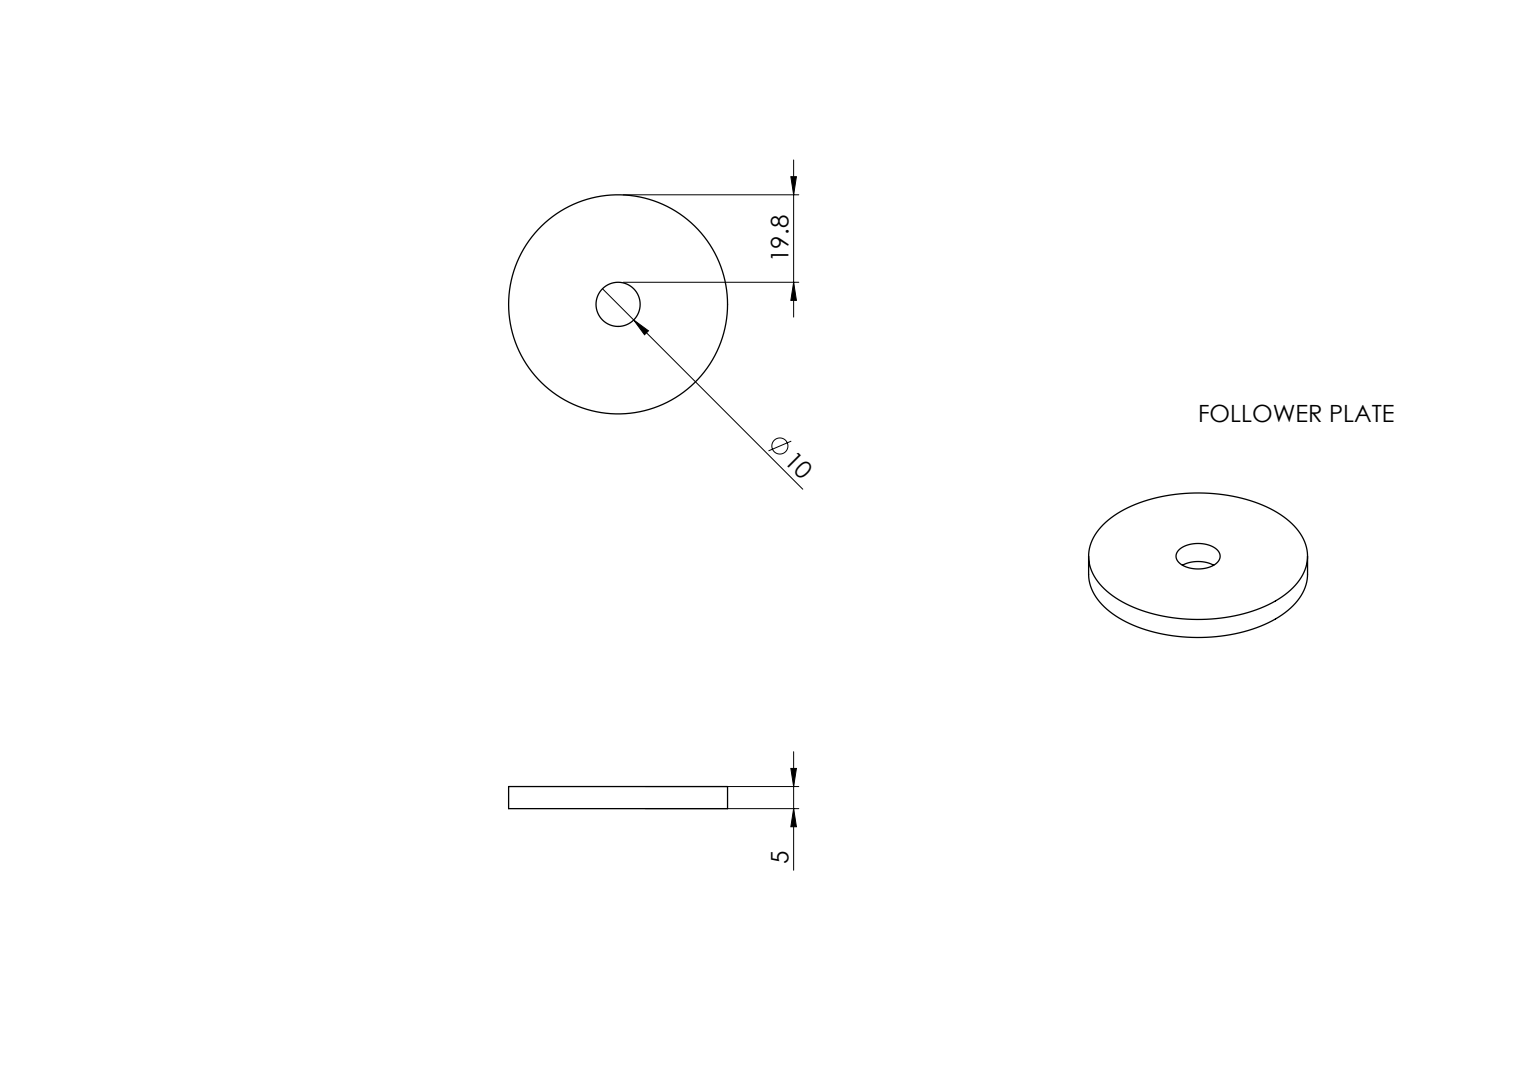
ISO-10303-21;
HEADER;
FILE_DESCRIPTION (('STEP AP214'),
    '1' );
FILE_NAME ('follower plate.step',
    '2026-10-31T03:36:27',
    ( '' ),
    ( '' ),
    'SwSTEP 2.0',
    'SolidWorks 2026',
    '' );
FILE_SCHEMA (( 'AUTOMOTIVE_DESIGN' ));
ENDSEC;

DATA;
#186=CARTESIAN_POINT ( 'NONE',  ( 0.000000000000000000, 148.0000000000000000, 0.000000000000000000 ) ) ;
#892=DIRECTION ( 'NONE',  ( 1.000000000000000000, 0.000000000000000000, 0.000000000000000000 ) ) ;
#1332=VECTOR ( 'NONE', #31249, 1000.000000000000000 ) ;
#1567=APPLICATION_CONTEXT ( 'automotive_design' ) ;
#1999=CLOSED_SHELL ( 'NONE', ( #16368, #12231, #10763, #12020, #10658, #28577 ) ) ;
#2419=AXIS2_PLACEMENT_3D ( 'NONE', #186, #17642, #35053 ) ;
#2606=ORIENTED_EDGE ( 'NONE', *, *, #4345, .F. ) ;
#2751=DIRECTION ( 'NONE',  ( 0.000000000000000000, 0.000000000000000000, -1.000000000000000000 ) ) ;
#3108=PRESENTATION_STYLE_ASSIGNMENT (( #5764 ) ) ;
#3154=CARTESIAN_POINT ( 'NONE',  ( 0.000000000000000000, 148.0000000000000000, -5.000000000000000888 ) ) ;
#3391=EDGE_CURVE ( 'NONE', #15520, #17083, #7946, .T. ) ;
#3436=AXIS2_PLACEMENT_3D ( 'NONE', #21969, #13622, #10578 ) ;
#3512=PRODUCT ( 'follower plate', 'follower plate', '', ( #4473 ) ) ;
#3678=EDGE_CURVE ( 'NONE', #35499, #36556, #26294, .T. ) ;
#3830=( GEOMETRIC_REPRESENTATION_CONTEXT ( 3 ) GLOBAL_UNCERTAINTY_ASSIGNED_CONTEXT ( ( #10847 ) ) GLOBAL_UNIT_ASSIGNED_CONTEXT ( ( #27171, #6708, #30204 ) ) REPRESENTATION_CONTEXT ( 'NONE', 'WORKASPACE' ) );
#4005=EDGE_CURVE ( 'NONE', #19287, #15548, #15251, .T. ) ;
#4007=ORIENTED_EDGE ( 'NONE', *, *, #23768, .F. ) ;
#4149=CIRCLE ( 'NONE', #8989, 5.000000000000000888 ) ;
#4345=EDGE_CURVE ( 'NONE', #35499, #15520, #10408, .T. ) ;
#4473=PRODUCT_CONTEXT ( 'NONE', #1567, 'mechanical' ) ;
#4527=SHAPE_REPRESENTATION ( 'follower plate', ( #17215 ), #16540 ) ;
#4651=DIRECTION ( 'NONE',  ( 0.000000000000000000, 0.000000000000000000, 1.000000000000000000 ) ) ;
#5261=CYLINDRICAL_SURFACE ( 'NONE', #3436, 5.000000000000000888 ) ;
#5315=LINE ( 'NONE', #16892, #20213 ) ;
#5752=ORIENTED_EDGE ( 'NONE', *, *, #7976, .F. ) ;
#5764=SURFACE_STYLE_USAGE ( .BOTH. , #34577 ) ;
#5780=CYLINDRICAL_SURFACE ( 'NONE', #25925, 24.80000000000000426 ) ;
#5837=CARTESIAN_POINT ( 'NONE',  ( 0.000000000000000000, 143.0000000000000000, 0.000000000000000000 ) ) ;
#5951=SURFACE_STYLE_FILL_AREA ( #23029 ) ;
#6046=CARTESIAN_POINT ( 'NONE',  ( 0.000000000000000000, 143.0000000000000000, -5.000000000000000888 ) ) ;
#6236=PRODUCT_DEFINITION_SHAPE ( 'NONE', 'NONE',  #37054 ) ;
#6285=DIRECTION ( 'NONE',  ( 0.000000000000000000, 0.000000000000000000, -1.000000000000000000 ) ) ;
#6655=ORIENTED_EDGE ( 'NONE', *, *, #4345, .T. ) ;
#6708=( NAMED_UNIT ( * ) PLANE_ANGLE_UNIT ( ) SI_UNIT ( $, .RADIAN. ) );
#6775=DIRECTION ( 'NONE',  ( 0.000000000000000000, 1.000000000000000000, 0.000000000000000000 ) ) ;
#7289=ORIENTED_EDGE ( 'NONE', *, *, #4005, .F. ) ;
#7513=MANIFOLD_SOLID_BREP ( 'Extrude-Thin1', #1999 ) ;
#7946=LINE ( 'NONE', #33719, #1332 ) ;
#7976=EDGE_CURVE ( 'NONE', #36216, #15548, #5315, .T. ) ;
#8069=COLOUR_RGB ( '',0.8941176470588234615, 0.8941176470588234615, 0.8941176470588234615 ) ;
#8268=FACE_OUTER_BOUND ( 'NONE', #23646, .T. ) ;
#8795=ORIENTED_EDGE ( 'NONE', *, *, #32424, .F. ) ;
#8806=( LENGTH_UNIT ( ) NAMED_UNIT ( * ) SI_UNIT ( .MILLI., .METRE. ) );
#8989=AXIS2_PLACEMENT_3D ( 'NONE', #29950, #18597, #33170 ) ;
#8991=( NAMED_UNIT ( * ) PLANE_ANGLE_UNIT ( ) SI_UNIT ( $, .RADIAN. ) );
#9205=EDGE_LOOP ( 'NONE', ( #23577, #31014, #20897, #8795 ) ) ;
#9458=CIRCLE ( 'NONE', #29444, 5.000000000000000888 ) ;
#9808=DIRECTION ( 'NONE',  ( -0.000000000000000000, -1.000000000000000000, -0.000000000000000000 ) ) ;
#9992=CARTESIAN_POINT ( 'NONE',  ( 0.000000000000000000, 148.0000000000000000, 0.000000000000000000 ) ) ;
#10237=ORIENTED_EDGE ( 'NONE', *, *, #3391, .T. ) ;
#10268=ORIENTED_EDGE ( 'NONE', *, *, #32424, .T. ) ;
#10369=CARTESIAN_POINT ( 'NONE',  ( 0.000000000000000000, 148.0000000000000000, 0.000000000000000000 ) ) ;
#10392=FACE_OUTER_BOUND ( 'NONE', #20693, .T. ) ;
#10408=CIRCLE ( 'NONE', #28551, 5.000000000000000888 ) ;
#10578=DIRECTION ( 'NONE',  ( 0.000000000000000000, 0.000000000000000000, -1.000000000000000000 ) ) ;
#10658=ADVANCED_FACE ( 'NONE', ( #36322 ), #27426, .T. ) ;
#10763=ADVANCED_FACE ( 'NONE', ( #36510, #32739 ), #35954, .T. ) ;
#10780=CARTESIAN_POINT ( 'NONE',  ( 0.000000000000000000, 143.0000000000000000, -24.80000000000000426 ) ) ;
#10847=UNCERTAINTY_MEASURE_WITH_UNIT (LENGTH_MEASURE( 1.000000000000000082E-05 ), #27171, 'distance_accuracy_value', 'NONE');
#11474=FACE_OUTER_BOUND ( 'NONE', #9205, .T. ) ;
#11740=VECTOR ( 'NONE', #29669, 1000.000000000000000 ) ;
#12020=ADVANCED_FACE ( 'NONE', ( #8268, #28346 ), #36871, .F. ) ;
#12161=DIRECTION ( 'NONE',  ( 0.000000000000000000, 1.000000000000000000, 0.000000000000000000 ) ) ;
#12231=ADVANCED_FACE ( 'NONE', ( #11474 ), #5780, .T. ) ;
#12385=EDGE_LOOP ( 'NONE', ( #5752, #24553, #10268, #37206 ) ) ;
#12416=AXIS2_PLACEMENT_3D ( 'NONE', #5837, #36923, #34642 ) ;
#12614=CARTESIAN_POINT ( 'NONE',  ( 0.000000000000000000, 148.0000000000000000, -24.80000000000000426 ) ) ;
#12653=DIRECTION ( 'NONE',  ( 0.000000000000000000, -0.000000000000000000, 1.000000000000000000 ) ) ;
#13177=LINE ( 'NONE', #12614, #11740 ) ;
#13178=EDGE_CURVE ( 'NONE', #17083, #36556, #4149, .T. ) ;
#13461=ORIENTED_EDGE ( 'NONE', *, *, #17015, .T. ) ;
#13622=DIRECTION ( 'NONE',  ( -0.000000000000000000, -1.000000000000000000, -0.000000000000000000 ) ) ;
#13740=( NAMED_UNIT ( * ) SI_UNIT ( $, .STERADIAN. ) SOLID_ANGLE_UNIT ( ) );
#13869=ORIENTED_EDGE ( 'NONE', *, *, #27231, .F. ) ;
#13986=AXIS2_PLACEMENT_3D ( 'NONE', #23540, #32245, #6285 ) ;
#14090=EDGE_LOOP ( 'NONE', ( #19838, #13461 ) ) ;
#14238=ADVANCED_BREP_SHAPE_REPRESENTATION ( '', ( #7513, #17215 ), #16540 ) ;
#14535=PRODUCT_DEFINITION_CONTEXT ( 'detailed design', #14628, 'design' ) ;
#14628=APPLICATION_CONTEXT ( 'automotive_design' ) ;
#14697=AXIS2_PLACEMENT_3D ( 'NONE', #9992, #6775, #12653 ) ;
#15045=ORIENTED_EDGE ( 'NONE', *, *, #13178, .F. ) ;
#15251=CIRCLE ( 'NONE', #21917, 24.80000000000000426 ) ;
#15520=VERTEX_POINT ( 'NONE', #3154 ) ;
#15548=VERTEX_POINT ( 'NONE', #34804 ) ;
#16047=CARTESIAN_POINT ( 'NONE',  ( 0.000000000000000000, 0.000000000000000000, 0.000000000000000000 ) ) ;
#16219=ORIENTED_EDGE ( 'NONE', *, *, #3678, .F. ) ;
#16368=ADVANCED_FACE ( 'NONE', ( #26369 ), #20701, .F. ) ;
#16428=ORIENTED_EDGE ( 'NONE', *, *, #13178, .T. ) ;
#16432=DIRECTION ( 'NONE',  ( 0.000000000000000000, 1.000000000000000000, 0.000000000000000000 ) ) ;
#16540=( GEOMETRIC_REPRESENTATION_CONTEXT ( 3 ) GLOBAL_UNCERTAINTY_ASSIGNED_CONTEXT ( ( #22239 ) ) GLOBAL_UNIT_ASSIGNED_CONTEXT ( ( #8806, #8991, #34397 ) ) REPRESENTATION_CONTEXT ( 'NONE', 'WORKASPACE' ) );
#16892=CARTESIAN_POINT ( 'NONE',  ( 3.037124061885436328E-15, 148.0000000000000000, 24.80000000000000426 ) ) ;
#17015=EDGE_CURVE ( 'NONE', #36216, #18565, #31526, .T. ) ;
#17083=VERTEX_POINT ( 'NONE', #6046 ) ;
#17215=AXIS2_PLACEMENT_3D ( 'NONE', #16047, #4651, #19645 ) ;
#17642=DIRECTION ( 'NONE',  ( 0.000000000000000000, 1.000000000000000000, 0.000000000000000000 ) ) ;
#17751=ORIENTED_EDGE ( 'NONE', *, *, #3391, .F. ) ;
#18565=VERTEX_POINT ( 'NONE', #29175 ) ;
#18597=DIRECTION ( 'NONE',  ( 0.000000000000000000, 1.000000000000000000, 0.000000000000000000 ) ) ;
#18725=EDGE_CURVE ( 'NONE', #18565, #36216, #28438, .T. ) ;
#19287=VERTEX_POINT ( 'NONE', #10780 ) ;
#19471=DIRECTION ( 'NONE',  ( 0.000000000000000000, -0.000000000000000000, 1.000000000000000000 ) ) ;
#19645=DIRECTION ( 'NONE',  ( 1.000000000000000000, 0.000000000000000000, 0.000000000000000000 ) ) ;
#19822=CARTESIAN_POINT ( 'NONE',  ( 0.000000000000000000, 143.0000000000000000, 0.000000000000000000 ) ) ;
#19838=ORIENTED_EDGE ( 'NONE', *, *, #18725, .T. ) ;
#20213=VECTOR ( 'NONE', #28431, 1000.000000000000000 ) ;
#20693=EDGE_LOOP ( 'NONE', ( #16219, #6655, #10237, #4007 ) ) ;
#20701=CYLINDRICAL_SURFACE ( 'NONE', #13986, 5.000000000000000888 ) ;
#20897=ORIENTED_EDGE ( 'NONE', *, *, #25595, .T. ) ;
#20899=DIRECTION ( 'NONE',  ( 0.000000000000000000, 0.000000000000000000, 1.000000000000000000 ) ) ;
#20930=AXIS2_PLACEMENT_3D ( 'NONE', #19822, #37035, #33837 ) ;
#21023=CARTESIAN_POINT ( 'NONE',  ( 6.123233995736767268E-16, 148.0000000000000000, 5.000000000000000888 ) ) ;
#21198=CARTESIAN_POINT ( 'NONE',  ( 0.000000000000000000, 143.0000000000000000, 0.000000000000000000 ) ) ;
#21571=DIRECTION ( 'NONE',  ( 0.000000000000000000, 1.000000000000000000, 0.000000000000000000 ) ) ;
#21917=AXIS2_PLACEMENT_3D ( 'NONE', #21198, #21571, #892 ) ;
#21944=DIRECTION ( 'NONE',  ( 0.000000000000000000, 0.000000000000000000, -1.000000000000000000 ) ) ;
#21969=CARTESIAN_POINT ( 'NONE',  ( 0.000000000000000000, 148.0000000000000000, 0.000000000000000000 ) ) ;
#22239=UNCERTAINTY_MEASURE_WITH_UNIT (LENGTH_MEASURE( 1.000000000000000082E-05 ), #8806, 'distance_accuracy_value', 'NONE');
#22607=EDGE_LOOP ( 'NONE', ( #13869, #2606 ) ) ;
#23029=FILL_AREA_STYLE ('',( #37411 ) ) ;
#23045=CARTESIAN_POINT ( 'NONE',  ( 0.000000000000000000, 148.0000000000000000, 0.000000000000000000 ) ) ;
#23095=DIRECTION ( 'NONE',  ( -0.000000000000000000, -1.000000000000000000, -0.000000000000000000 ) ) ;
#23336=ORIENTED_EDGE ( 'NONE', *, *, #3678, .T. ) ;
#23540=CARTESIAN_POINT ( 'NONE',  ( 0.000000000000000000, 148.0000000000000000, 0.000000000000000000 ) ) ;
#23577=ORIENTED_EDGE ( 'NONE', *, *, #17015, .F. ) ;
#23646=EDGE_LOOP ( 'NONE', ( #7289, #34064 ) ) ;
#23768=EDGE_CURVE ( 'NONE', #36556, #17083, #27569, .T. ) ;
#24553=ORIENTED_EDGE ( 'NONE', *, *, #18725, .F. ) ;
#25038=UNCERTAINTY_MEASURE_WITH_UNIT (LENGTH_MEASURE( 1.000000000000000082E-05 ), #33824, 'distance_accuracy_value', 'NONE');
#25595=EDGE_CURVE ( 'NONE', #15548, #19287, #26972, .T. ) ;
#25877=DIRECTION ( 'NONE',  ( -0.000000000000000000, -1.000000000000000000, -0.000000000000000000 ) ) ;
#25925=AXIS2_PLACEMENT_3D ( 'NONE', #23045, #25877, #2751 ) ;
#26294=LINE ( 'NONE', #37475, #27357 ) ;
#26369=FACE_OUTER_BOUND ( 'NONE', #32838, .T. ) ;
#26972=CIRCLE ( 'NONE', #20930, 24.80000000000000426 ) ;
#27171=( LENGTH_UNIT ( ) NAMED_UNIT ( * ) SI_UNIT ( .MILLI., .METRE. ) );
#27231=EDGE_CURVE ( 'NONE', #15520, #35499, #9458, .T. ) ;
#27357=VECTOR ( 'NONE', #23095, 1000.000000000000000 ) ;
#27426=CYLINDRICAL_SURFACE ( 'NONE', #31055, 24.80000000000000426 ) ;
#27569=CIRCLE ( 'NONE', #12416, 5.000000000000000888 ) ;
#27738=AXIS2_PLACEMENT_3D ( 'NONE', #27797, #16432, #19471 ) ;
#27797=CARTESIAN_POINT ( 'NONE',  ( 0.000000000000000000, 143.0000000000000000, 0.000000000000000000 ) ) ;
#27804=DIRECTION ( 'NONE',  ( 0.000000000000000000, 1.000000000000000000, 0.000000000000000000 ) ) ;
#27957=CARTESIAN_POINT ( 'NONE',  ( 6.123233995736767268E-16, 143.0000000000000000, 5.000000000000000888 ) ) ;
#27986=DIRECTION ( 'NONE',  ( 0.000000000000000000, 0.000000000000000000, 1.000000000000000000 ) ) ;
#28129=( NAMED_UNIT ( * ) PLANE_ANGLE_UNIT ( ) SI_UNIT ( $, .RADIAN. ) );
#28346=FACE_BOUND ( 'NONE', #36827, .T. ) ;
#28431=DIRECTION ( 'NONE',  ( -0.000000000000000000, -1.000000000000000000, -0.000000000000000000 ) ) ;
#28438=CIRCLE ( 'NONE', #2419, 24.80000000000000426 ) ;
#28551=AXIS2_PLACEMENT_3D ( 'NONE', #33487, #27804, #27986 ) ;
#28577=ADVANCED_FACE ( 'NONE', ( #10392 ), #5261, .F. ) ;
#29175=CARTESIAN_POINT ( 'NONE',  ( 0.000000000000000000, 148.0000000000000000, -24.80000000000000426 ) ) ;
#29223=MECHANICAL_DESIGN_GEOMETRIC_PRESENTATION_REPRESENTATION('',(#30481),#3830);
#29444=AXIS2_PLACEMENT_3D ( 'NONE', #35091, #12161, #20899 ) ;
#29669=DIRECTION ( 'NONE',  ( -0.000000000000000000, -1.000000000000000000, -0.000000000000000000 ) ) ;
#29881=SHAPE_DEFINITION_REPRESENTATION ( #6236, #4527 ) ;
#29950=CARTESIAN_POINT ( 'NONE',  ( 0.000000000000000000, 143.0000000000000000, 0.000000000000000000 ) ) ;
#30015=SHAPE_REPRESENTATION_RELATIONSHIP ( 'NONE' , 'NONE' ,  #4527, #14238 ) ;
#30204=( NAMED_UNIT ( * ) SI_UNIT ( $, .STERADIAN. ) SOLID_ANGLE_UNIT ( ) );
#30481=STYLED_ITEM ( 'NONE', ( #3108 ), #14238 ) ;
#31014=ORIENTED_EDGE ( 'NONE', *, *, #7976, .T. ) ;
#31055=AXIS2_PLACEMENT_3D ( 'NONE', #10369, #9808, #21944 ) ;
#31116=MECHANICAL_DESIGN_GEOMETRIC_PRESENTATION_REPRESENTATION('',(#37159),#35337);
#31249=DIRECTION ( 'NONE',  ( -0.000000000000000000, -1.000000000000000000, -0.000000000000000000 ) ) ;
#31461=CARTESIAN_POINT ( 'NONE',  ( 0.000000000000000000, 148.0000000000000000, 0.000000000000000000 ) ) ;
#31526=CIRCLE ( 'NONE', #34554, 24.80000000000000426 ) ;
#31829=DIRECTION ( 'NONE',  ( 1.000000000000000000, 0.000000000000000000, 0.000000000000000000 ) ) ;
#31863=ORIENTED_EDGE ( 'NONE', *, *, #23768, .T. ) ;
#32015=DIRECTION ( 'NONE',  ( 0.000000000000000000, 1.000000000000000000, 0.000000000000000000 ) ) ;
#32245=DIRECTION ( 'NONE',  ( -0.000000000000000000, -1.000000000000000000, -0.000000000000000000 ) ) ;
#32424=EDGE_CURVE ( 'NONE', #18565, #19287, #13177, .T. ) ;
#32739=FACE_BOUND ( 'NONE', #22607, .T. ) ;
#32838=EDGE_LOOP ( 'NONE', ( #37347, #23336, #15045, #17751 ) ) ;
#33170=DIRECTION ( 'NONE',  ( 0.000000000000000000, 0.000000000000000000, 1.000000000000000000 ) ) ;
#33487=CARTESIAN_POINT ( 'NONE',  ( 0.000000000000000000, 148.0000000000000000, 0.000000000000000000 ) ) ;
#33719=CARTESIAN_POINT ( 'NONE',  ( 0.000000000000000000, 148.0000000000000000, -5.000000000000000888 ) ) ;
#33824=( LENGTH_UNIT ( ) NAMED_UNIT ( * ) SI_UNIT ( .MILLI., .METRE. ) );
#33837=DIRECTION ( 'NONE',  ( 1.000000000000000000, 0.000000000000000000, 0.000000000000000000 ) ) ;
#34064=ORIENTED_EDGE ( 'NONE', *, *, #25595, .F. ) ;
#34253=CARTESIAN_POINT ( 'NONE',  ( 3.037124061885436328E-15, 148.0000000000000000, 24.80000000000000426 ) ) ;
#34397=( NAMED_UNIT ( * ) SI_UNIT ( $, .STERADIAN. ) SOLID_ANGLE_UNIT ( ) );
#34554=AXIS2_PLACEMENT_3D ( 'NONE', #31461, #32015, #31829 ) ;
#34577=SURFACE_SIDE_STYLE ('',( #5951 ) ) ;
#34642=DIRECTION ( 'NONE',  ( 0.000000000000000000, 0.000000000000000000, 1.000000000000000000 ) ) ;
#34804=CARTESIAN_POINT ( 'NONE',  ( 3.037124061885436328E-15, 143.0000000000000000, 24.80000000000000426 ) ) ;
#35053=DIRECTION ( 'NONE',  ( 1.000000000000000000, 0.000000000000000000, 0.000000000000000000 ) ) ;
#35091=CARTESIAN_POINT ( 'NONE',  ( 0.000000000000000000, 148.0000000000000000, 0.000000000000000000 ) ) ;
#35337=( GEOMETRIC_REPRESENTATION_CONTEXT ( 3 ) GLOBAL_UNCERTAINTY_ASSIGNED_CONTEXT ( ( #25038 ) ) GLOBAL_UNIT_ASSIGNED_CONTEXT ( ( #33824, #28129, #13740 ) ) REPRESENTATION_CONTEXT ( 'NONE', 'WORKASPACE' ) );
#35499=VERTEX_POINT ( 'NONE', #21023 ) ;
#35947=PRODUCT_DEFINITION_FORMATION_WITH_SPECIFIED_SOURCE ( 'ANY', '', #3512, .NOT_KNOWN. ) ;
#35954=PLANE ( 'NONE',  #14697 ) ;
#36216=VERTEX_POINT ( 'NONE', #34253 ) ;
#36322=FACE_OUTER_BOUND ( 'NONE', #12385, .T. ) ;
#36510=FACE_OUTER_BOUND ( 'NONE', #14090, .T. ) ;
#36556=VERTEX_POINT ( 'NONE', #27957 ) ;
#36827=EDGE_LOOP ( 'NONE', ( #16428, #31863 ) ) ;
#36871=PLANE ( 'NONE',  #27738 ) ;
#36923=DIRECTION ( 'NONE',  ( 0.000000000000000000, 1.000000000000000000, 0.000000000000000000 ) ) ;
#37035=DIRECTION ( 'NONE',  ( 0.000000000000000000, 1.000000000000000000, 0.000000000000000000 ) ) ;
#37054=PRODUCT_DEFINITION ( 'UNKNOWN', '', #35947, #14535 ) ;
#37159=STYLED_ITEM('',(#37556),#7513);
#37206=ORIENTED_EDGE ( 'NONE', *, *, #4005, .T. ) ;
#37347=ORIENTED_EDGE ( 'NONE', *, *, #27231, .T. ) ;
#37411=FILL_AREA_STYLE_COLOUR ( '', #8069 ) ;
#37475=CARTESIAN_POINT ( 'NONE',  ( 6.123233995736767268E-16, 148.0000000000000000, 5.000000000000000888 ) ) ;
#37550=COLOUR_RGB('Off White',0.89,0.88,0.83);
#37551=FILL_AREA_STYLE_COLOUR('',#37550);
#37552=FILL_AREA_STYLE('',(#37551));
#37553=SURFACE_STYLE_FILL_AREA(#37552);
#37554=SURFACE_SIDE_STYLE('',(#37553));
#37555=SURFACE_STYLE_USAGE(.BOTH.,#37554);
#37556=PRESENTATION_STYLE_ASSIGNMENT((#37555));
ENDSEC;
END-ISO-10303-21;
